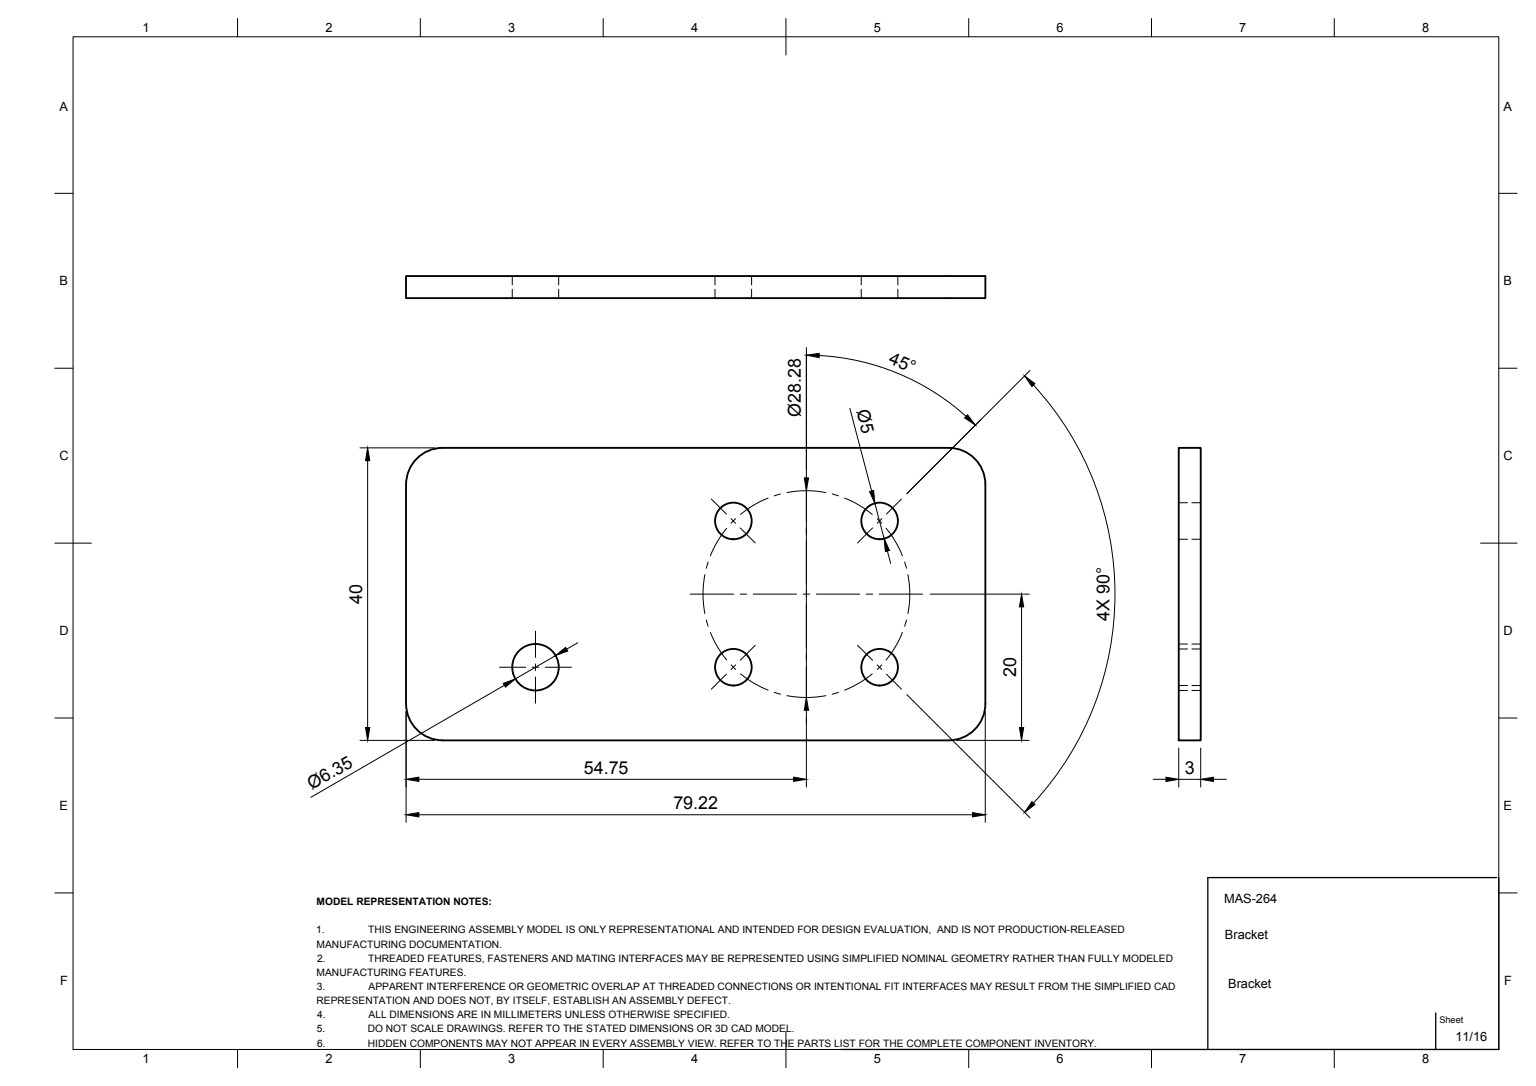
ISO-10303-21;
HEADER;
/* Generated by software containing ST-Developer
 * from STEP Tools, Inc. (www.steptools.com) 
 */

FILE_DESCRIPTION(
/* description */ (''),
/* implementation_level */ '2;1');

FILE_NAME(
/* name */ 'Bracket.step',
/* time_stamp */ '2026-10-12T15:37:13-07:00',
/* author */ (''),
/* organization */ (''),
/* preprocessor_version */ 'ST-DEVELOPER v20.2',
/* originating_system */ 'Autodesk Translation Framework v15.15.0.0',
/* authorisation */ '');

FILE_SCHEMA (('AUTOMOTIVE_DESIGN { 1 0 10303 214 3 1 1 }'));
ENDSEC;

DATA;
#10=MECHANICAL_DESIGN_GEOMETRIC_PRESENTATION_REPRESENTATION('',(#356),#36460);
#117=SHAPE_REPRESENTATION_RELATIONSHIP('SRR','None',#36529,#130);
#130=ADVANCED_BREP_SHAPE_REPRESENTATION('',(#388),#36458);
#253=FACE_BOUND('',#2356,.T.);
#254=FACE_BOUND('',#2357,.T.);
#255=FACE_BOUND('',#2358,.T.);
#256=FACE_BOUND('',#2359,.T.);
#257=FACE_BOUND('',#2360,.T.);
#258=FACE_BOUND('',#2362,.T.);
#259=FACE_BOUND('',#2363,.T.);
#260=FACE_BOUND('',#2364,.T.);
#261=FACE_BOUND('',#2365,.T.);
#262=FACE_BOUND('',#2366,.T.);
#356=STYLED_ITEM('',(#36596),#388);
#388=MANIFOLD_SOLID_BREP('Body1',#11292);
#693=PLANE('',#12378);
#694=PLANE('',#12382);
#695=PLANE('',#12386);
#696=PLANE('',#12390);
#697=PLANE('',#12391);
#698=PLANE('',#12392);
#1607=FACE_OUTER_BOUND('',#2342,.T.);
#1608=FACE_OUTER_BOUND('',#2343,.T.);
#1609=FACE_OUTER_BOUND('',#2344,.T.);
#1610=FACE_OUTER_BOUND('',#2345,.T.);
#1611=FACE_OUTER_BOUND('',#2346,.T.);
#1612=FACE_OUTER_BOUND('',#2347,.T.);
#1613=FACE_OUTER_BOUND('',#2348,.T.);
#1614=FACE_OUTER_BOUND('',#2349,.T.);
#1615=FACE_OUTER_BOUND('',#2350,.T.);
#1616=FACE_OUTER_BOUND('',#2351,.T.);
#1617=FACE_OUTER_BOUND('',#2352,.T.);
#1618=FACE_OUTER_BOUND('',#2353,.T.);
#1619=FACE_OUTER_BOUND('',#2354,.T.);
#1620=FACE_OUTER_BOUND('',#2355,.T.);
#1621=FACE_OUTER_BOUND('',#2361,.T.);
#2342=EDGE_LOOP('',(#10268,#10269,#10270,#10271));
#2343=EDGE_LOOP('',(#10272,#10273,#10274,#10275));
#2344=EDGE_LOOP('',(#10276,#10277,#10278,#10279));
#2345=EDGE_LOOP('',(#10280,#10281,#10282,#10283));
#2346=EDGE_LOOP('',(#10284,#10285,#10286,#10287));
#2347=EDGE_LOOP('',(#10288,#10289,#10290,#10291));
#2348=EDGE_LOOP('',(#10292,#10293,#10294,#10295));
#2349=EDGE_LOOP('',(#10296,#10297,#10298,#10299));
#2350=EDGE_LOOP('',(#10300,#10301,#10302,#10303));
#2351=EDGE_LOOP('',(#10304,#10305,#10306,#10307));
#2352=EDGE_LOOP('',(#10308,#10309,#10310,#10311));
#2353=EDGE_LOOP('',(#10312,#10313,#10314,#10315));
#2354=EDGE_LOOP('',(#10316,#10317,#10318,#10319));
#2355=EDGE_LOOP('',(#10320,#10321,#10322,#10323,#10324,#10325,#10326,#10327));
#2356=EDGE_LOOP('',(#10328));
#2357=EDGE_LOOP('',(#10329));
#2358=EDGE_LOOP('',(#10330));
#2359=EDGE_LOOP('',(#10331));
#2360=EDGE_LOOP('',(#10332));
#2361=EDGE_LOOP('',(#10333,#10334,#10335,#10336,#10337,#10338,#10339,#10340));
#2362=EDGE_LOOP('',(#10341));
#2363=EDGE_LOOP('',(#10342));
#2364=EDGE_LOOP('',(#10343));
#2365=EDGE_LOOP('',(#10344));
#2366=EDGE_LOOP('',(#10345));
#3287=LINE('',#36264,#4233);
#3288=LINE('',#36270,#4234);
#3289=LINE('',#36276,#4235);
#3290=LINE('',#36282,#4236);
#3291=LINE('',#36288,#4237);
#3292=LINE('',#36295,#4238);
#3293=LINE('',#36298,#4239);
#3294=LINE('',#36301,#4240);
#3295=LINE('',#36303,#4241);
#3296=LINE('',#36304,#4242);
#3297=LINE('',#36310,#4243);
#3298=LINE('',#36313,#4244);
#3299=LINE('',#36315,#4245);
#3300=LINE('',#36316,#4246);
#3301=LINE('',#36322,#4247);
#3302=LINE('',#36325,#4248);
#3303=LINE('',#36327,#4249);
#3304=LINE('',#36328,#4250);
#3305=LINE('',#36334,#4251);
#3306=LINE('',#36336,#4252);
#3307=LINE('',#36337,#4253);
#4233=VECTOR('',#15184,2.50000000000001);
#4234=VECTOR('',#15191,2.50000000000001);
#4235=VECTOR('',#15198,3.17500000000003);
#4236=VECTOR('',#15205,2.50000000000001);
#4237=VECTOR('',#15212,2.50000000000001);
#4238=VECTOR('',#15219,10.);
#4239=VECTOR('',#15222,10.);
#4240=VECTOR('',#15225,10.);
#4241=VECTOR('',#15226,10.);
#4242=VECTOR('',#15227,10.);
#4243=VECTOR('',#15234,10.);
#4244=VECTOR('',#15237,10.);
#4245=VECTOR('',#15238,10.);
#4246=VECTOR('',#15239,10.);
#4247=VECTOR('',#15246,10.);
#4248=VECTOR('',#15249,10.);
#4249=VECTOR('',#15250,10.);
#4250=VECTOR('',#15251,10.);
#4251=VECTOR('',#15258,10.);
#4252=VECTOR('',#15261,10.);
#4253=VECTOR('',#15262,10.);
#4567=CIRCLE('',#12361,2.50000000000001);
#4568=CIRCLE('',#12362,2.50000000000001);
#4569=CIRCLE('',#12364,2.50000000000001);
#4570=CIRCLE('',#12365,2.50000000000001);
#4571=CIRCLE('',#12367,3.17500000000003);
#4572=CIRCLE('',#12368,3.17500000000003);
#4573=CIRCLE('',#12370,2.50000000000001);
#4574=CIRCLE('',#12371,2.50000000000001);
#4575=CIRCLE('',#12373,2.50000000000001);
#4576=CIRCLE('',#12374,2.50000000000001);
#4577=CIRCLE('',#12376,4.99999999999993);
#4578=CIRCLE('',#12377,4.99999999999993);
#4579=CIRCLE('',#12380,4.99999999999993);
#4580=CIRCLE('',#12381,4.99999999999993);
#4581=CIRCLE('',#12384,5.);
#4582=CIRCLE('',#12385,5.);
#4583=CIRCLE('',#12388,5.);
#4584=CIRCLE('',#12389,5.);
#5605=VERTEX_POINT('',#36261);
#5606=VERTEX_POINT('',#36263);
#5607=VERTEX_POINT('',#36267);
#5608=VERTEX_POINT('',#36269);
#5609=VERTEX_POINT('',#36273);
#5610=VERTEX_POINT('',#36275);
#5611=VERTEX_POINT('',#36279);
#5612=VERTEX_POINT('',#36281);
#5613=VERTEX_POINT('',#36285);
#5614=VERTEX_POINT('',#36287);
#5615=VERTEX_POINT('',#36291);
#5616=VERTEX_POINT('',#36292);
#5617=VERTEX_POINT('',#36294);
#5618=VERTEX_POINT('',#36296);
#5619=VERTEX_POINT('',#36300);
#5620=VERTEX_POINT('',#36302);
#5621=VERTEX_POINT('',#36306);
#5622=VERTEX_POINT('',#36308);
#5623=VERTEX_POINT('',#36312);
#5624=VERTEX_POINT('',#36314);
#5625=VERTEX_POINT('',#36318);
#5626=VERTEX_POINT('',#36320);
#5627=VERTEX_POINT('',#36324);
#5628=VERTEX_POINT('',#36326);
#5629=VERTEX_POINT('',#36330);
#5630=VERTEX_POINT('',#36332);
#7165=EDGE_CURVE('',#5605,#5605,#4567,.T.);
#7166=EDGE_CURVE('',#5605,#5606,#3287,.T.);
#7167=EDGE_CURVE('',#5606,#5606,#4568,.T.);
#7168=EDGE_CURVE('',#5607,#5607,#4569,.T.);
#7169=EDGE_CURVE('',#5607,#5608,#3288,.T.);
#7170=EDGE_CURVE('',#5608,#5608,#4570,.T.);
#7171=EDGE_CURVE('',#5609,#5609,#4571,.T.);
#7172=EDGE_CURVE('',#5609,#5610,#3289,.T.);
#7173=EDGE_CURVE('',#5610,#5610,#4572,.T.);
#7174=EDGE_CURVE('',#5611,#5611,#4573,.T.);
#7175=EDGE_CURVE('',#5611,#5612,#3290,.T.);
#7176=EDGE_CURVE('',#5612,#5612,#4574,.T.);
#7177=EDGE_CURVE('',#5613,#5613,#4575,.T.);
#7178=EDGE_CURVE('',#5613,#5614,#3291,.T.);
#7179=EDGE_CURVE('',#5614,#5614,#4576,.T.);
#7180=EDGE_CURVE('',#5615,#5616,#4577,.T.);
#7181=EDGE_CURVE('',#5615,#5617,#3292,.T.);
#7182=EDGE_CURVE('',#5618,#5617,#4578,.T.);
#7183=EDGE_CURVE('',#5616,#5618,#3293,.T.);
#7184=EDGE_CURVE('',#5619,#5616,#3294,.T.);
#7185=EDGE_CURVE('',#5620,#5618,#3295,.T.);
#7186=EDGE_CURVE('',#5619,#5620,#3296,.T.);
#7187=EDGE_CURVE('',#5619,#5621,#4579,.T.);
#7188=EDGE_CURVE('',#5622,#5620,#4580,.T.);
#7189=EDGE_CURVE('',#5621,#5622,#3297,.T.);
#7190=EDGE_CURVE('',#5623,#5621,#3298,.T.);
#7191=EDGE_CURVE('',#5624,#5622,#3299,.T.);
#7192=EDGE_CURVE('',#5623,#5624,#3300,.T.);
#7193=EDGE_CURVE('',#5623,#5625,#4581,.T.);
#7194=EDGE_CURVE('',#5626,#5624,#4582,.T.);
#7195=EDGE_CURVE('',#5625,#5626,#3301,.T.);
#7196=EDGE_CURVE('',#5627,#5625,#3302,.T.);
#7197=EDGE_CURVE('',#5628,#5626,#3303,.T.);
#7198=EDGE_CURVE('',#5627,#5628,#3304,.T.);
#7199=EDGE_CURVE('',#5627,#5629,#4583,.T.);
#7200=EDGE_CURVE('',#5630,#5628,#4584,.T.);
#7201=EDGE_CURVE('',#5629,#5630,#3305,.T.);
#7202=EDGE_CURVE('',#5615,#5629,#3306,.T.);
#7203=EDGE_CURVE('',#5617,#5630,#3307,.T.);
#10268=ORIENTED_EDGE('',*,*,#7165,.F.);
#10269=ORIENTED_EDGE('',*,*,#7166,.T.);
#10270=ORIENTED_EDGE('',*,*,#7167,.F.);
#10271=ORIENTED_EDGE('',*,*,#7166,.F.);
#10272=ORIENTED_EDGE('',*,*,#7168,.F.);
#10273=ORIENTED_EDGE('',*,*,#7169,.T.);
#10274=ORIENTED_EDGE('',*,*,#7170,.F.);
#10275=ORIENTED_EDGE('',*,*,#7169,.F.);
#10276=ORIENTED_EDGE('',*,*,#7171,.F.);
#10277=ORIENTED_EDGE('',*,*,#7172,.T.);
#10278=ORIENTED_EDGE('',*,*,#7173,.F.);
#10279=ORIENTED_EDGE('',*,*,#7172,.F.);
#10280=ORIENTED_EDGE('',*,*,#7174,.F.);
#10281=ORIENTED_EDGE('',*,*,#7175,.T.);
#10282=ORIENTED_EDGE('',*,*,#7176,.F.);
#10283=ORIENTED_EDGE('',*,*,#7175,.F.);
#10284=ORIENTED_EDGE('',*,*,#7177,.F.);
#10285=ORIENTED_EDGE('',*,*,#7178,.T.);
#10286=ORIENTED_EDGE('',*,*,#7179,.F.);
#10287=ORIENTED_EDGE('',*,*,#7178,.F.);
#10288=ORIENTED_EDGE('',*,*,#7180,.F.);
#10289=ORIENTED_EDGE('',*,*,#7181,.T.);
#10290=ORIENTED_EDGE('',*,*,#7182,.F.);
#10291=ORIENTED_EDGE('',*,*,#7183,.F.);
#10292=ORIENTED_EDGE('',*,*,#7184,.T.);
#10293=ORIENTED_EDGE('',*,*,#7183,.T.);
#10294=ORIENTED_EDGE('',*,*,#7185,.F.);
#10295=ORIENTED_EDGE('',*,*,#7186,.F.);
#10296=ORIENTED_EDGE('',*,*,#7187,.F.);
#10297=ORIENTED_EDGE('',*,*,#7186,.T.);
#10298=ORIENTED_EDGE('',*,*,#7188,.F.);
#10299=ORIENTED_EDGE('',*,*,#7189,.F.);
#10300=ORIENTED_EDGE('',*,*,#7190,.T.);
#10301=ORIENTED_EDGE('',*,*,#7189,.T.);
#10302=ORIENTED_EDGE('',*,*,#7191,.F.);
#10303=ORIENTED_EDGE('',*,*,#7192,.F.);
#10304=ORIENTED_EDGE('',*,*,#7193,.F.);
#10305=ORIENTED_EDGE('',*,*,#7192,.T.);
#10306=ORIENTED_EDGE('',*,*,#7194,.F.);
#10307=ORIENTED_EDGE('',*,*,#7195,.F.);
#10308=ORIENTED_EDGE('',*,*,#7196,.T.);
#10309=ORIENTED_EDGE('',*,*,#7195,.T.);
#10310=ORIENTED_EDGE('',*,*,#7197,.F.);
#10311=ORIENTED_EDGE('',*,*,#7198,.F.);
#10312=ORIENTED_EDGE('',*,*,#7199,.F.);
#10313=ORIENTED_EDGE('',*,*,#7198,.T.);
#10314=ORIENTED_EDGE('',*,*,#7200,.F.);
#10315=ORIENTED_EDGE('',*,*,#7201,.F.);
#10316=ORIENTED_EDGE('',*,*,#7202,.T.);
#10317=ORIENTED_EDGE('',*,*,#7201,.T.);
#10318=ORIENTED_EDGE('',*,*,#7203,.F.);
#10319=ORIENTED_EDGE('',*,*,#7181,.F.);
#10320=ORIENTED_EDGE('',*,*,#7202,.F.);
#10321=ORIENTED_EDGE('',*,*,#7180,.T.);
#10322=ORIENTED_EDGE('',*,*,#7184,.F.);
#10323=ORIENTED_EDGE('',*,*,#7187,.T.);
#10324=ORIENTED_EDGE('',*,*,#7190,.F.);
#10325=ORIENTED_EDGE('',*,*,#7193,.T.);
#10326=ORIENTED_EDGE('',*,*,#7196,.F.);
#10327=ORIENTED_EDGE('',*,*,#7199,.T.);
#10328=ORIENTED_EDGE('',*,*,#7177,.T.);
#10329=ORIENTED_EDGE('',*,*,#7174,.T.);
#10330=ORIENTED_EDGE('',*,*,#7171,.T.);
#10331=ORIENTED_EDGE('',*,*,#7168,.T.);
#10332=ORIENTED_EDGE('',*,*,#7165,.T.);
#10333=ORIENTED_EDGE('',*,*,#7203,.T.);
#10334=ORIENTED_EDGE('',*,*,#7200,.T.);
#10335=ORIENTED_EDGE('',*,*,#7197,.T.);
#10336=ORIENTED_EDGE('',*,*,#7194,.T.);
#10337=ORIENTED_EDGE('',*,*,#7191,.T.);
#10338=ORIENTED_EDGE('',*,*,#7188,.T.);
#10339=ORIENTED_EDGE('',*,*,#7185,.T.);
#10340=ORIENTED_EDGE('',*,*,#7182,.T.);
#10341=ORIENTED_EDGE('',*,*,#7179,.T.);
#10342=ORIENTED_EDGE('',*,*,#7176,.T.);
#10343=ORIENTED_EDGE('',*,*,#7173,.T.);
#10344=ORIENTED_EDGE('',*,*,#7170,.T.);
#10345=ORIENTED_EDGE('',*,*,#7167,.T.);
#10638=CYLINDRICAL_SURFACE('',#12360,2.50000000000001);
#10639=CYLINDRICAL_SURFACE('',#12363,2.50000000000001);
#10640=CYLINDRICAL_SURFACE('',#12366,3.17500000000003);
#10641=CYLINDRICAL_SURFACE('',#12369,2.50000000000001);
#10642=CYLINDRICAL_SURFACE('',#12372,2.50000000000001);
#10643=CYLINDRICAL_SURFACE('',#12375,4.99999999999993);
#10644=CYLINDRICAL_SURFACE('',#12379,4.99999999999993);
#10645=CYLINDRICAL_SURFACE('',#12383,5.);
#10646=CYLINDRICAL_SURFACE('',#12387,5.);
#11228=ADVANCED_FACE('',(#1607),#10638,.F.);
#11229=ADVANCED_FACE('',(#1608),#10639,.F.);
#11230=ADVANCED_FACE('',(#1609),#10640,.F.);
#11231=ADVANCED_FACE('',(#1610),#10641,.F.);
#11232=ADVANCED_FACE('',(#1611),#10642,.F.);
#11233=ADVANCED_FACE('',(#1612),#10643,.T.);
#11234=ADVANCED_FACE('',(#1613),#693,.T.);
#11235=ADVANCED_FACE('',(#1614),#10644,.T.);
#11236=ADVANCED_FACE('',(#1615),#694,.T.);
#11237=ADVANCED_FACE('',(#1616),#10645,.T.);
#11238=ADVANCED_FACE('',(#1617),#695,.T.);
#11239=ADVANCED_FACE('',(#1618),#10646,.T.);
#11240=ADVANCED_FACE('',(#1619),#696,.T.);
#11241=ADVANCED_FACE('',(#1620,#253,#254,#255,#256,#257),#697,.T.);
#11242=ADVANCED_FACE('',(#1621,#258,#259,#260,#261,#262),#698,.F.);
#11292=CLOSED_SHELL('',(#11228,#11229,#11230,#11231,#11232,#11233,#11234,
#11235,#11236,#11237,#11238,#11239,#11240,#11241,#11242));
#12359=AXIS2_PLACEMENT_3D('',#36259,#15178,#15179);
#12360=AXIS2_PLACEMENT_3D('',#36260,#15180,#15181);
#12361=AXIS2_PLACEMENT_3D('',#36262,#15182,#15183);
#12362=AXIS2_PLACEMENT_3D('',#36265,#15185,#15186);
#12363=AXIS2_PLACEMENT_3D('',#36266,#15187,#15188);
#12364=AXIS2_PLACEMENT_3D('',#36268,#15189,#15190);
#12365=AXIS2_PLACEMENT_3D('',#36271,#15192,#15193);
#12366=AXIS2_PLACEMENT_3D('',#36272,#15194,#15195);
#12367=AXIS2_PLACEMENT_3D('',#36274,#15196,#15197);
#12368=AXIS2_PLACEMENT_3D('',#36277,#15199,#15200);
#12369=AXIS2_PLACEMENT_3D('',#36278,#15201,#15202);
#12370=AXIS2_PLACEMENT_3D('',#36280,#15203,#15204);
#12371=AXIS2_PLACEMENT_3D('',#36283,#15206,#15207);
#12372=AXIS2_PLACEMENT_3D('',#36284,#15208,#15209);
#12373=AXIS2_PLACEMENT_3D('',#36286,#15210,#15211);
#12374=AXIS2_PLACEMENT_3D('',#36289,#15213,#15214);
#12375=AXIS2_PLACEMENT_3D('',#36290,#15215,#15216);
#12376=AXIS2_PLACEMENT_3D('',#36293,#15217,#15218);
#12377=AXIS2_PLACEMENT_3D('',#36297,#15220,#15221);
#12378=AXIS2_PLACEMENT_3D('',#36299,#15223,#15224);
#12379=AXIS2_PLACEMENT_3D('',#36305,#15228,#15229);
#12380=AXIS2_PLACEMENT_3D('',#36307,#15230,#15231);
#12381=AXIS2_PLACEMENT_3D('',#36309,#15232,#15233);
#12382=AXIS2_PLACEMENT_3D('',#36311,#15235,#15236);
#12383=AXIS2_PLACEMENT_3D('',#36317,#15240,#15241);
#12384=AXIS2_PLACEMENT_3D('',#36319,#15242,#15243);
#12385=AXIS2_PLACEMENT_3D('',#36321,#15244,#15245);
#12386=AXIS2_PLACEMENT_3D('',#36323,#15247,#15248);
#12387=AXIS2_PLACEMENT_3D('',#36329,#15252,#15253);
#12388=AXIS2_PLACEMENT_3D('',#36331,#15254,#15255);
#12389=AXIS2_PLACEMENT_3D('',#36333,#15256,#15257);
#12390=AXIS2_PLACEMENT_3D('',#36335,#15259,#15260);
#12391=AXIS2_PLACEMENT_3D('',#36338,#15263,#15264);
#12392=AXIS2_PLACEMENT_3D('',#36339,#15265,#15266);
#15178=DIRECTION('axis',(0.,0.,1.));
#15179=DIRECTION('refdir',(1.,0.,0.));
#15180=DIRECTION('center_axis',(0.,0.,-1.));
#15181=DIRECTION('ref_axis',(1.,0.,0.));
#15182=DIRECTION('center_axis',(0.,0.,-1.));
#15183=DIRECTION('ref_axis',(1.,0.,0.));
#15184=DIRECTION('',(0.,0.,-1.));
#15185=DIRECTION('center_axis',(0.,0.,1.));
#15186=DIRECTION('ref_axis',(1.,0.,0.));
#15187=DIRECTION('center_axis',(0.,0.,-1.));
#15188=DIRECTION('ref_axis',(1.,0.,0.));
#15189=DIRECTION('center_axis',(0.,0.,-1.));
#15190=DIRECTION('ref_axis',(1.,0.,0.));
#15191=DIRECTION('',(0.,0.,-1.));
#15192=DIRECTION('center_axis',(0.,0.,1.));
#15193=DIRECTION('ref_axis',(1.,0.,0.));
#15194=DIRECTION('center_axis',(0.,0.,-1.));
#15195=DIRECTION('ref_axis',(1.,0.,0.));
#15196=DIRECTION('center_axis',(0.,-1.13806187638273E-62,-1.));
#15197=DIRECTION('ref_axis',(1.,0.,0.));
#15198=DIRECTION('',(0.,0.,-1.));
#15199=DIRECTION('center_axis',(0.,1.13806187638273E-62,1.));
#15200=DIRECTION('ref_axis',(1.,0.,0.));
#15201=DIRECTION('center_axis',(0.,0.,-1.));
#15202=DIRECTION('ref_axis',(1.,0.,0.));
#15203=DIRECTION('center_axis',(0.,0.,-1.));
#15204=DIRECTION('ref_axis',(1.,0.,0.));
#15205=DIRECTION('',(0.,0.,-1.));
#15206=DIRECTION('center_axis',(0.,0.,1.));
#15207=DIRECTION('ref_axis',(1.,0.,0.));
#15208=DIRECTION('center_axis',(0.,0.,-1.));
#15209=DIRECTION('ref_axis',(1.,0.,0.));
#15210=DIRECTION('center_axis',(0.,0.,-1.));
#15211=DIRECTION('ref_axis',(1.,0.,0.));
#15212=DIRECTION('',(0.,0.,-1.));
#15213=DIRECTION('center_axis',(0.,0.,1.));
#15214=DIRECTION('ref_axis',(1.,0.,0.));
#15215=DIRECTION('center_axis',(0.,0.,-1.));
#15216=DIRECTION('ref_axis',(-1.,1.42108547152022E-14,0.));
#15217=DIRECTION('center_axis',(-1.98364274472311E-31,1.40137711657962E-17,
1.));
#15218=DIRECTION('ref_axis',(-1.,1.42108547152022E-14,-3.97511940521531E-31));
#15219=DIRECTION('',(0.,0.,-1.));
#15220=DIRECTION('center_axis',(1.98364274472311E-31,-1.40137711657962E-17,
-1.));
#15221=DIRECTION('ref_axis',(-1.,1.42108547152022E-14,-3.97511940521531E-31));
#15222=DIRECTION('',(0.,0.,-1.));
#15223=DIRECTION('center_axis',(2.368475785867E-15,-1.,0.));
#15224=DIRECTION('ref_axis',(-1.,-2.368475785867E-15,4.56151843855735E-49));
#15225=DIRECTION('',(-1.,-2.368475785867E-15,4.56151843855735E-49));
#15226=DIRECTION('',(-1.,-2.368475785867E-15,4.56151843855735E-49));
#15227=DIRECTION('',(0.,0.,-1.));
#15228=DIRECTION('center_axis',(0.,0.,-1.));
#15229=DIRECTION('ref_axis',(8.88178419700138E-16,-1.,0.));
#15230=DIRECTION('center_axis',(-5.36441819030946E-47,1.60253698400202E-32,
1.));
#15231=DIRECTION('ref_axis',(8.88178419700138E-16,-1.,1.60253698400202E-32));
#15232=DIRECTION('center_axis',(5.36441819030946E-47,-1.60253698400202E-32,
-1.));
#15233=DIRECTION('ref_axis',(8.88178419700138E-16,-1.,1.60253698400202E-32));
#15234=DIRECTION('',(0.,0.,-1.));
#15235=DIRECTION('center_axis',(1.,-6.41527552355446E-17,0.));
#15236=DIRECTION('ref_axis',(-6.41527552355446E-17,-1.,6.85517916879725E-33));
#15237=DIRECTION('',(-6.41527552355446E-17,-1.,6.85517916879725E-33));
#15238=DIRECTION('',(-6.41527552355446E-17,-1.,6.85517916879725E-33));
#15239=DIRECTION('',(0.,0.,-1.));
#15240=DIRECTION('center_axis',(0.,0.,-1.));
#15241=DIRECTION('ref_axis',(1.,1.4210854715202E-14,0.));
#15242=DIRECTION('center_axis',(-5.55111512312578E-17,-3.88267476788466E-31,
1.));
#15243=DIRECTION('ref_axis',(1.,1.4210854715202E-14,5.55111512312578E-17));
#15244=DIRECTION('center_axis',(5.55111512312578E-17,3.88267476788466E-31,
-1.));
#15245=DIRECTION('ref_axis',(1.,1.4210854715202E-14,5.55111512312578E-17));
#15246=DIRECTION('',(0.,0.,-1.));
#15247=DIRECTION('center_axis',(0.,1.,0.));
#15248=DIRECTION('ref_axis',(1.,0.,1.8503717077086E-17));
#15249=DIRECTION('',(1.,0.,1.8503717077086E-17));
#15250=DIRECTION('',(1.,0.,1.8503717077086E-17));
#15251=DIRECTION('',(0.,0.,-1.));
#15252=DIRECTION('center_axis',(0.,0.,-1.));
#15253=DIRECTION('ref_axis',(0.,1.,0.));
#15254=DIRECTION('center_axis',(-2.77555756156289E-17,2.8027542331593E-17,
1.));
#15255=DIRECTION('ref_axis',(0.,1.,-2.8027542331593E-17));
#15256=DIRECTION('center_axis',(2.77555756156289E-17,-2.8027542331593E-17,
-1.));
#15257=DIRECTION('ref_axis',(0.,1.,-2.8027542331593E-17));
#15258=DIRECTION('',(0.,0.,-1.));
#15259=DIRECTION('center_axis',(-1.,-3.20763776177723E-16,0.));
#15260=DIRECTION('ref_axis',(-3.20763776177723E-16,1.,-1.30015623442515E-17));
#15261=DIRECTION('',(-3.20763776177723E-16,1.,-1.30015623442515E-17));
#15262=DIRECTION('',(-3.20763776177723E-16,1.,-1.30015623442515E-17));
#15263=DIRECTION('center_axis',(-1.8503717077086E-17,0.,1.));
#15264=DIRECTION('ref_axis',(1.,0.,1.8503717077086E-17));
#15265=DIRECTION('center_axis',(-1.8503717077086E-17,0.,1.));
#15266=DIRECTION('ref_axis',(1.,0.,1.8503717077086E-17));
#36259=CARTESIAN_POINT('',(0.,0.,0.));
#36260=CARTESIAN_POINT('Origin',(10.,493.005151372827,-9.99999999999999));
#36261=CARTESIAN_POINT('',(7.49999999999999,493.005151372827,-9.99999999999999));
#36262=CARTESIAN_POINT('Origin',(10.,493.005151372827,-9.99999999999999));
#36263=CARTESIAN_POINT('',(7.49999999999999,493.005151372827,-13.));
#36264=CARTESIAN_POINT('',(7.49999999999999,493.005151372827,-9.99999999999999));
#36265=CARTESIAN_POINT('Origin',(10.,493.005151372827,-13.));
#36266=CARTESIAN_POINT('Origin',(-10.,473.005151372827,-9.99999999999999));
#36267=CARTESIAN_POINT('',(-12.5,473.005151372827,-9.99999999999999));
#36268=CARTESIAN_POINT('Origin',(-10.,473.005151372827,-9.99999999999999));
#36269=CARTESIAN_POINT('',(-12.5,473.005151372827,-13.));
#36270=CARTESIAN_POINT('',(-12.5,473.005151372827,-9.99999999999999));
#36271=CARTESIAN_POINT('Origin',(-10.,473.005151372827,-13.));
#36272=CARTESIAN_POINT('Origin',(-9.99999999999998,520.056498641762,-9.99999999999999));
#36273=CARTESIAN_POINT('',(-13.175,520.056498641762,-9.99999999999999));
#36274=CARTESIAN_POINT('Origin',(-9.99999999999998,520.056498641762,-9.99999999999999));
#36275=CARTESIAN_POINT('',(-13.175,520.056498641762,-13.));
#36276=CARTESIAN_POINT('',(-13.175,520.056498641762,-9.99999999999999));
#36277=CARTESIAN_POINT('Origin',(-9.99999999999998,520.056498641762,-13.));
#36278=CARTESIAN_POINT('Origin',(-10.,493.005151372827,-9.99999999999999));
#36279=CARTESIAN_POINT('',(-12.5,493.005151372827,-9.99999999999999));
#36280=CARTESIAN_POINT('Origin',(-10.,493.005151372827,-9.99999999999999));
#36281=CARTESIAN_POINT('',(-12.5,493.005151372827,-13.));
#36282=CARTESIAN_POINT('',(-12.5,493.005151372827,-9.99999999999999));
#36283=CARTESIAN_POINT('Origin',(-10.,493.005151372827,-13.));
#36284=CARTESIAN_POINT('Origin',(10.,473.005151372827,-9.99999999999999));
#36285=CARTESIAN_POINT('',(7.49999999999999,473.005151372827,-9.99999999999999));
#36286=CARTESIAN_POINT('Origin',(10.,473.005151372827,-9.99999999999999));
#36287=CARTESIAN_POINT('',(7.49999999999999,473.005151372827,-13.));
#36288=CARTESIAN_POINT('',(7.49999999999999,473.005151372827,-9.99999999999999));
#36289=CARTESIAN_POINT('Origin',(10.,473.005151372827,-13.));
#36290=CARTESIAN_POINT('Origin',(-15.,463.536269734217,-9.99999999999999));
#36291=CARTESIAN_POINT('',(-20.,463.536269734217,-9.99999999999999));
#36292=CARTESIAN_POINT('',(-15.,458.536269734217,-9.99999999999999));
#36293=CARTESIAN_POINT('Origin',(-15.,463.536269734217,-9.99999999999999));
#36294=CARTESIAN_POINT('',(-20.,463.536269734217,-13.));
#36295=CARTESIAN_POINT('',(-20.,463.536269734217,-9.99999999999999));
#36296=CARTESIAN_POINT('',(-15.,458.536269734217,-13.));
#36297=CARTESIAN_POINT('Origin',(-15.,463.536269734217,-13.));
#36298=CARTESIAN_POINT('',(-15.,458.536269734217,-9.99999999999999));
#36299=CARTESIAN_POINT('Origin',(15.,458.536269734217,-9.99999999999999));
#36300=CARTESIAN_POINT('',(15.,458.536269734217,-9.99999999999999));
#36301=CARTESIAN_POINT('',(15.,458.536269734217,-9.99999999999999));
#36302=CARTESIAN_POINT('',(15.,458.536269734217,-13.));
#36303=CARTESIAN_POINT('',(15.,458.536269734217,-13.));
#36304=CARTESIAN_POINT('',(15.,458.536269734217,-9.99999999999999));
#36305=CARTESIAN_POINT('Origin',(15.,463.536269734217,-9.99999999999999));
#36306=CARTESIAN_POINT('',(19.9999999999999,463.536269734217,-9.99999999999999));
#36307=CARTESIAN_POINT('Origin',(15.,463.536269734217,-9.99999999999999));
#36308=CARTESIAN_POINT('',(19.9999999999999,463.536269734217,-13.));
#36309=CARTESIAN_POINT('Origin',(15.,463.536269734217,-13.));
#36310=CARTESIAN_POINT('',(19.9999999999999,463.536269734217,-9.99999999999999));
#36311=CARTESIAN_POINT('Origin',(20.,532.759985569887,-9.99999999999999));
#36312=CARTESIAN_POINT('',(20.,532.759985569887,-9.99999999999999));
#36313=CARTESIAN_POINT('',(20.,532.759985569887,-9.99999999999999));
#36314=CARTESIAN_POINT('',(20.,532.759985569887,-13.));
#36315=CARTESIAN_POINT('',(20.,532.759985569887,-13.));
#36316=CARTESIAN_POINT('',(20.,532.759985569887,-9.99999999999999));
#36317=CARTESIAN_POINT('Origin',(15.,532.759985569887,-9.99999999999999));
#36318=CARTESIAN_POINT('',(15.,537.759985569887,-9.99999999999999));
#36319=CARTESIAN_POINT('Origin',(15.,532.759985569887,-9.99999999999999));
#36320=CARTESIAN_POINT('',(15.,537.759985569887,-13.));
#36321=CARTESIAN_POINT('Origin',(15.,532.759985569887,-13.));
#36322=CARTESIAN_POINT('',(15.,537.759985569887,-9.99999999999999));
#36323=CARTESIAN_POINT('Origin',(-15.,537.759985569887,-9.99999999999999));
#36324=CARTESIAN_POINT('',(-15.,537.759985569887,-9.99999999999999));
#36325=CARTESIAN_POINT('',(-15.,537.759985569887,-9.99999999999999));
#36326=CARTESIAN_POINT('',(-15.,537.759985569887,-13.));
#36327=CARTESIAN_POINT('',(-15.,537.759985569887,-13.));
#36328=CARTESIAN_POINT('',(-15.,537.759985569887,-9.99999999999999));
#36329=CARTESIAN_POINT('Origin',(-15.,532.759985569887,-9.99999999999999));
#36330=CARTESIAN_POINT('',(-20.,532.759985569887,-9.99999999999999));
#36331=CARTESIAN_POINT('Origin',(-15.,532.759985569887,-9.99999999999999));
#36332=CARTESIAN_POINT('',(-20.,532.759985569887,-13.));
#36333=CARTESIAN_POINT('Origin',(-15.,532.759985569887,-13.));
#36334=CARTESIAN_POINT('',(-20.,532.759985569887,-9.99999999999999));
#36335=CARTESIAN_POINT('Origin',(-20.,463.536269734217,-9.99999999999999));
#36336=CARTESIAN_POINT('',(-20.,463.536269734217,-9.99999999999999));
#36337=CARTESIAN_POINT('',(-20.,463.536269734217,-13.));
#36338=CARTESIAN_POINT('Origin',(-7.58590136239051E-15,498.148127652052,
-9.99999999999999));
#36339=CARTESIAN_POINT('Origin',(-7.58590136239051E-15,498.148127652052,
-13.));
#36442=UNCERTAINTY_MEASURE_WITH_UNIT(LENGTH_MEASURE(0.01),#36461,
'DISTANCE_ACCURACY_VALUE',
'Maximum model space distance between geometric entities at asserted c
onnectivities');
#36444=UNCERTAINTY_MEASURE_WITH_UNIT(LENGTH_MEASURE(0.01),#36461,
'DISTANCE_ACCURACY_VALUE',
'Maximum model space distance between geometric entities at asserted c
onnectivities');
#36458=(
GEOMETRIC_REPRESENTATION_CONTEXT(3)
GLOBAL_UNCERTAINTY_ASSIGNED_CONTEXT((#36442))
GLOBAL_UNIT_ASSIGNED_CONTEXT((#36461,#36463,#36464))
REPRESENTATION_CONTEXT('','3D')
);
#36460=(
GEOMETRIC_REPRESENTATION_CONTEXT(3)
GLOBAL_UNCERTAINTY_ASSIGNED_CONTEXT((#36444))
GLOBAL_UNIT_ASSIGNED_CONTEXT((#36461,#36463,#36464))
REPRESENTATION_CONTEXT('','3D')
);
#36461=(
LENGTH_UNIT()
NAMED_UNIT(*)
SI_UNIT(.MILLI.,.METRE.)
);
#36463=(
NAMED_UNIT(*)
PLANE_ANGLE_UNIT()
SI_UNIT($,.RADIAN.)
);
#36464=(
NAMED_UNIT(*)
SI_UNIT($,.STERADIAN.)
SOLID_ANGLE_UNIT()
);
#36478=SHAPE_DEFINITION_REPRESENTATION(#36498,#36529);
#36498=PRODUCT_DEFINITION_SHAPE('',$,#36545);
#36529=SHAPE_REPRESENTATION('',(#12359),#36458);
#36531=PRODUCT_DEFINITION_CONTEXT('part definition',#36578,'design');
#36545=PRODUCT_DEFINITION('Bracket','Bracket',#36560,#36531);
#36560=PRODUCT_DEFINITION_FORMATION('',$,#36593);
#36578=APPLICATION_CONTEXT(
'Core Data for Automotive Mechanical Design Process');
#36579=PRODUCT_CONTEXT('part definition',#36578,'mechanical');
#36593=PRODUCT('Bracket','Bracket',$,(#36579));
#36596=PRESENTATION_STYLE_ASSIGNMENT((#36601));
#36601=SURFACE_STYLE_USAGE(.BOTH.,#36606);
#36606=SURFACE_SIDE_STYLE('',(#36611));
#36611=SURFACE_STYLE_FILL_AREA(#36616);
#36616=FILL_AREA_STYLE('Opaque(160,160,160)',(#36621));
#36621=FILL_AREA_STYLE_COLOUR('Opaque(160,160,160)',#36626);
#36626=COLOUR_RGB('Opaque(160,160,160)', 0.09019608, 0.27058824, 0.51372549);
ENDSEC;
END-ISO-10303-21;
